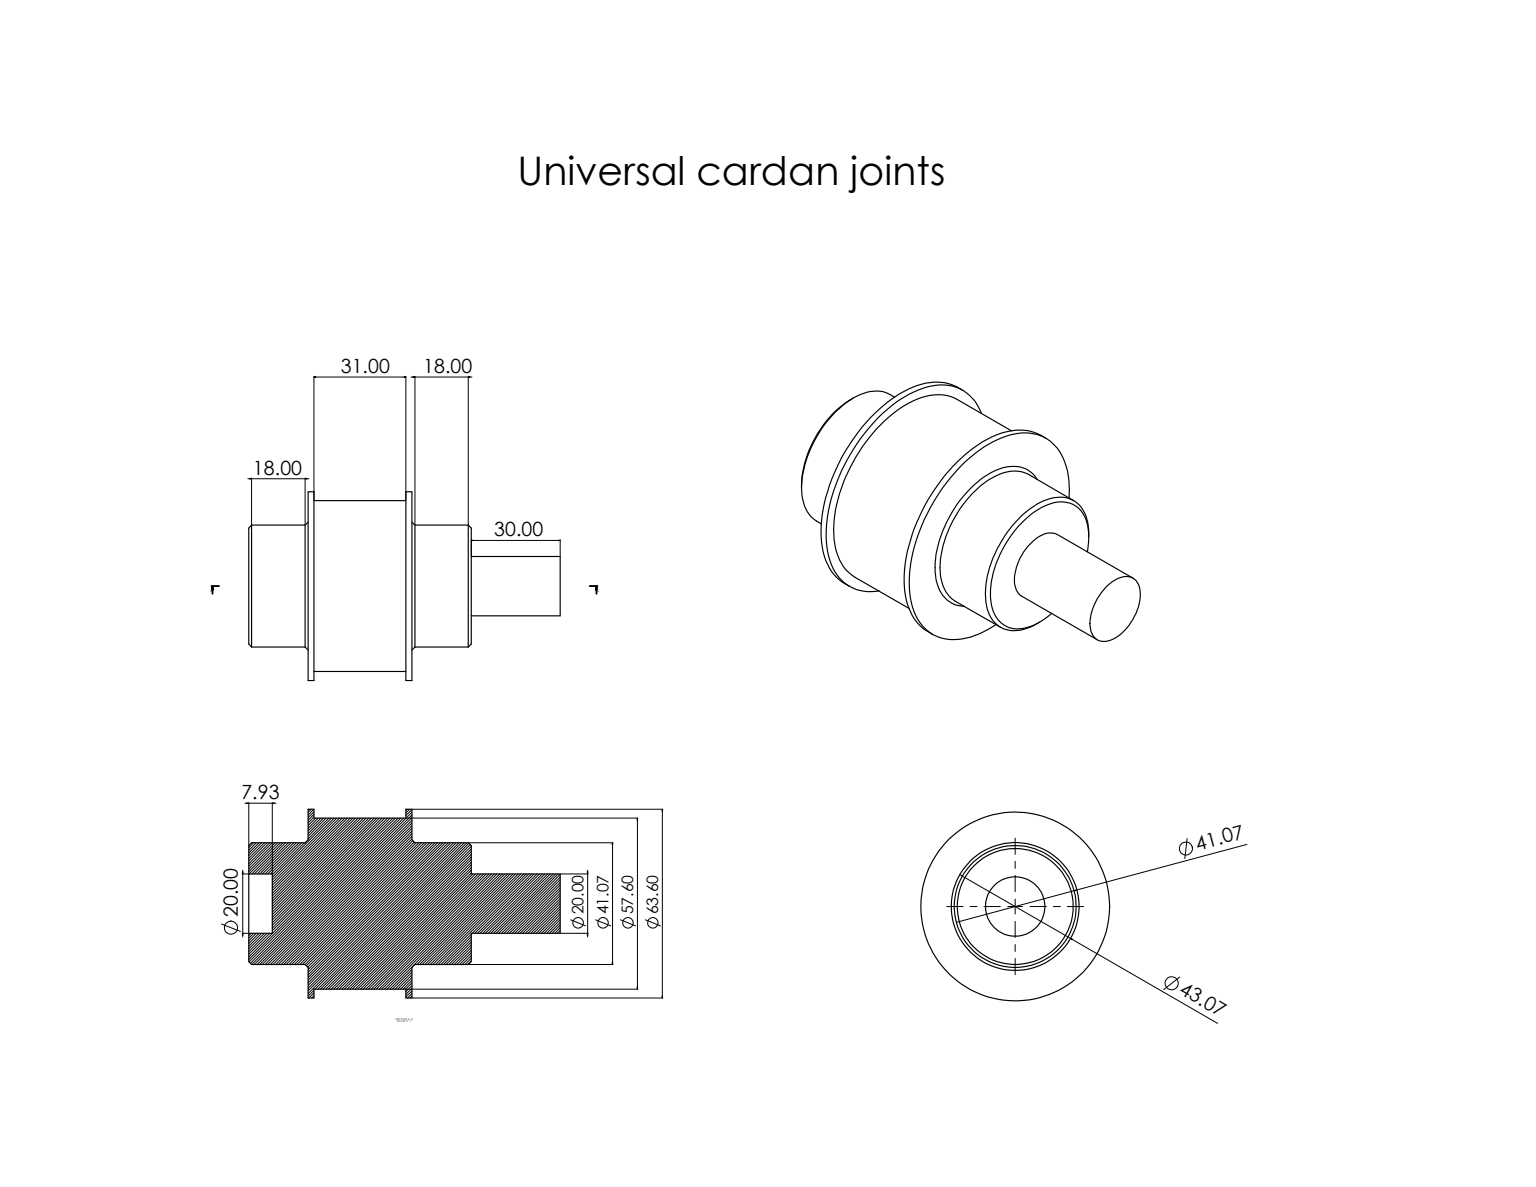
ISO-10303-21;
HEADER;
FILE_DESCRIPTION (('STEP AP214'),
    '1' );
FILE_NAME ('Universal cardan joints.step',
    '2026-10-27T19:20:31',
    ( '' ),
    ( '' ),
    'SwSTEP 2.0',
    'SolidWorks 2025',
    '' );
FILE_SCHEMA (( 'AUTOMOTIVE_DESIGN' ));
ENDSEC;

DATA;
#22=DIRECTION ( 'NONE',  ( 0.000000000000000000, 0.000000000000000000, 1.000000000000000000 ) ) ;
#28=ORIENTED_EDGE ( 'NONE', *, *, #15718, .T. ) ;
#34=DIRECTION ( 'NONE',  ( 0.000000000000000000, 0.000000000000000000, 1.000000000000000000 ) ) ;
#74=DIRECTION ( 'NONE',  ( -1.000000000000000000, 0.000000000000000000, 0.000000000000000000 ) ) ;
#91=ORIENTED_EDGE ( 'NONE', *, *, #1926, .F. ) ;
#97=VECTOR ( 'NONE', #21456, 1000.000000000000000 ) ;
#195=PRODUCT ( 'Universal cardan joints', 'Universal cardan joints', '', ( #26348 ) ) ;
#244=AXIS2_PLACEMENT_3D ( 'NONE', #3180, #21532, #25538 ) ;
#277=AXIS2_PLACEMENT_3D ( 'NONE', #11873, #9385, #1278 ) ;
#288=ORIENTED_EDGE ( 'NONE', *, *, #2639, .F. ) ;
#299=DIRECTION ( 'NONE',  ( -1.000000000000000000, -0.000000000000000000, -0.000000000000000000 ) ) ;
#421=CARTESIAN_POINT ( 'NONE',  ( -370.0000000000001137, -4.857225732735059864E-14, 0.000000000000000000 ) ) ;
#440=CARTESIAN_POINT ( 'NONE',  ( -295.0000000000000568, -4.857225732735059864E-14, 0.000000000000000000 ) ) ;
#464=AXIS2_PLACEMENT_3D ( 'NONE', #3688, #20320, #23901 ) ;
#478=DIRECTION ( 'NONE',  ( 0.000000000000000000, 0.000000000000000000, -1.000000000000000000 ) ) ;
#495=VERTEX_POINT ( 'NONE', #11725 ) ;
#573=DIRECTION ( 'NONE',  ( -1.000000000000000000, 0.000000000000000000, -0.000000000000000000 ) ) ;
#612=ADVANCED_FACE ( 'NONE', ( #6031 ), #23234, .T. ) ;
#783=CARTESIAN_POINT ( 'NONE',  ( -314.0000000000000568, -4.857225732735059864E-14, 0.000000000000000000 ) ) ;
#811=LINE ( 'NONE', #8516, #13626 ) ;
#825=( NAMED_UNIT ( * ) SI_UNIT ( $, .STERADIAN. ) SOLID_ANGLE_UNIT ( ) );
#827=ORIENTED_EDGE ( 'NONE', *, *, #8764, .F. ) ;
#862=VERTEX_POINT ( 'NONE', #20801 ) ;
#941=DIRECTION ( 'NONE',  ( -0.7071067811865302533, 0.000000000000000000, 0.7071067811865646702 ) ) ;
#984=ORIENTED_EDGE ( 'NONE', *, *, #22744, .T. ) ;
#996=DIRECTION ( 'NONE',  ( 0.000000000000000000, 0.000000000000000000, -1.000000000000000000 ) ) ;
#1025=EDGE_CURVE ( 'NONE', #20774, #23054, #12596, .T. ) ;
#1113=ORIENTED_EDGE ( 'NONE', *, *, #21755, .F. ) ;
#1121=PRODUCT_DEFINITION_CONTEXT ( 'detailed design', #16139, 'design' ) ;
#1241=ORIENTED_EDGE ( 'NONE', *, *, #9230, .F. ) ;
#1257=DIRECTION ( 'NONE',  ( 1.000000000000000000, 0.000000000000000000, 0.000000000000000000 ) ) ;
#1278=DIRECTION ( 'NONE',  ( 0.000000000000000000, 0.000000000000000000, -1.000000000000000000 ) ) ;
#1284=PLANE ( 'NONE',  #7860 ) ;
#1298=CARTESIAN_POINT ( 'NONE',  ( -296.0000000000000000, -4.857225732735059864E-14, 0.000000000000000000 ) ) ;
#1340=AXIS2_PLACEMENT_3D ( 'NONE', #8100, #26229, #11702 ) ;
#1341=CARTESIAN_POINT ( 'NONE',  ( -315.0000000000000568, -4.857225732735059864E-14, 0.000000000000000000 ) ) ;
#1377=ORIENTED_EDGE ( 'NONE', *, *, #13860, .T. ) ;
#1381=AXIS2_PLACEMENT_3D ( 'NONE', #11675, #9306, #19800 ) ;
#1389=CARTESIAN_POINT ( 'NONE',  ( -317.0000000000000568, -4.857225732735059864E-14, -31.79780246617542616 ) ) ;
#1404=DIRECTION ( 'NONE',  ( -1.000000000000000000, 0.000000000000000000, 0.000000000000000000 ) ) ;
#1425=VERTEX_POINT ( 'NONE', #2470 ) ;
#1458=DIRECTION ( 'NONE',  ( 0.000000000000000000, 0.000000000000000000, 1.000000000000000000 ) ) ;
#1507=CARTESIAN_POINT ( 'NONE',  ( -317.0000000000000568, -4.857225732735059864E-14, 0.000000000000000000 ) ) ;
#1570=UNCERTAINTY_MEASURE_WITH_UNIT (LENGTH_MEASURE( 1.000000000000000082E-05 ), #17119, 'distance_accuracy_value', 'NONE');
#1574=AXIS2_PLACEMENT_3D ( 'NONE', #23163, #13295, #7298 ) ;
#1578=CARTESIAN_POINT ( 'NONE',  ( -265.0000000000000000, -4.857225732735059864E-14, 10.00000000000000000 ) ) ;
#1579=DIRECTION ( 'NONE',  ( 0.7071067811865500152, 8.659560562354903276E-17, 0.7071067811865451302 ) ) ;
#1608=CARTESIAN_POINT ( 'NONE',  ( -362.0709805440841365, -4.734761052820324085E-14, -10.00000000000004796 ) ) ;
#1686=AXIS2_PLACEMENT_3D ( 'NONE', #17256, #9399, #13145 ) ;
#1695=CARTESIAN_POINT ( 'NONE',  ( -317.0000000000000568, -4.857225732735059864E-14, 0.000000000000000000 ) ) ;
#1704=CARTESIAN_POINT ( 'NONE',  ( -362.0709805440841365, -4.605747634845933236E-14, -20.53474504356812247 ) ) ;
#1740=EDGE_CURVE ( 'NONE', #20774, #862, #9363, .T. ) ;
#1766=AXIS2_PLACEMENT_3D ( 'NONE', #25196, #2714, #11077 ) ;
#1881=CARTESIAN_POINT ( 'NONE',  ( -295.0000000000000568, -4.734761052820324716E-14, -9.999999999999996447 ) ) ;
#1926=EDGE_CURVE ( 'NONE', #1425, #13433, #19253, .T. ) ;
#2016=ADVANCED_FACE ( 'NONE', ( #25514, #21508 ), #1284, .F. ) ;
#2084=AXIS2_PLACEMENT_3D ( 'NONE', #2569, #12809, #10684 ) ;
#2108=CYLINDRICAL_SURFACE ( 'NONE', #18230, 31.79780246617542616 ) ;
#2126=CIRCLE ( 'NONE', #10610, 20.53474504356812247 ) ;
#2127=ORIENTED_EDGE ( 'NONE', *, *, #14586, .T. ) ;
#2190=AXIS2_PLACEMENT_3D ( 'NONE', #6287, #4316, #22000 ) ;
#2213=DIRECTION ( 'NONE',  ( 1.000000000000000000, 0.000000000000000000, 0.000000000000000000 ) ) ;
#2326=LINE ( 'NONE', #18553, #4936 ) ;
#2385=DIRECTION ( 'NONE',  ( 0.000000000000000000, 0.000000000000000000, -1.000000000000000000 ) ) ;
#2390=DIRECTION ( 'NONE',  ( 0.000000000000000000, 0.000000000000000000, 1.000000000000000000 ) ) ;
#2455=VERTEX_POINT ( 'NONE', #6167 ) ;
#2470=CARTESIAN_POINT ( 'NONE',  ( -351.0000000000000568, -4.857225732735059864E-14, 20.53474504356812247 ) ) ;
#2497=AXIS2_PLACEMENT_3D ( 'NONE', #14303, #74, #16164 ) ;
#2564=FACE_OUTER_BOUND ( 'NONE', #16654, .T. ) ;
#2569=CARTESIAN_POINT ( 'NONE',  ( -362.0709805440841365, -4.857225732735059864E-14, 0.000000000000000000 ) ) ;
#2604=VECTOR ( 'NONE', #11874, 1000.000000000000000 ) ;
#2639=EDGE_CURVE ( 'NONE', #19072, #19714, #10510, .T. ) ;
#2697=VERTEX_POINT ( 'NONE', #10914 ) ;
#2709=DIRECTION ( 'NONE',  ( 1.000000000000000000, 0.000000000000000000, 0.000000000000000000 ) ) ;
#2714=DIRECTION ( 'NONE',  ( -1.000000000000000000, 0.000000000000000000, -0.000000000000000000 ) ) ;
#2830=ORIENTED_EDGE ( 'NONE', *, *, #4790, .T. ) ;
#2832=EDGE_LOOP ( 'NONE', ( #20393, #22553, #11090, #13813 ) ) ;
#2980=ADVANCED_FACE ( 'NONE', ( #9043 ), #15154, .F. ) ;
#3049=DIRECTION ( 'NONE',  ( -1.000000000000000000, -0.000000000000000000, -0.000000000000000000 ) ) ;
#3051=AXIS2_PLACEMENT_3D ( 'NONE', #24614, #22620, #12897 ) ;
#3055=DIRECTION ( 'NONE',  ( -1.000000000000000000, 0.000000000000000000, -0.000000000000000000 ) ) ;
#3081=AXIS2_PLACEMENT_3D ( 'NONE', #17412, #7552, #23664 ) ;
#3087=DIRECTION ( 'NONE',  ( -1.000000000000000000, 0.000000000000000000, 0.000000000000000000 ) ) ;
#3107=CARTESIAN_POINT ( 'NONE',  ( -315.0000000000000568, -4.857225732735059864E-14, 21.53474504356810115 ) ) ;
#3118=EDGE_CURVE ( 'NONE', #3897, #22348, #16821, .T. ) ;
#3146=EDGE_CURVE ( 'NONE', #26122, #19577, #26173, .T. ) ;
#3180=CARTESIAN_POINT ( 'NONE',  ( -370.0000000000001137, -4.857225732735059864E-14, 0.000000000000000000 ) ) ;
#3200=ORIENTED_EDGE ( 'NONE', *, *, #9955, .T. ) ;
#3209=CARTESIAN_POINT ( 'NONE',  ( -351.0000000000000568, -4.857225732735059864E-14, 0.000000000000000000 ) ) ;
#3237=CIRCLE ( 'NONE', #18086, 19.53474504356812602 ) ;
#3318=ORIENTED_EDGE ( 'NONE', *, *, #9230, .T. ) ;
#3329=EDGE_LOOP ( 'NONE', ( #14913, #4122, #9477, #25461 ) ) ;
#3365=DIRECTION ( 'NONE',  ( 1.000000000000000000, 0.000000000000000000, 0.000000000000000000 ) ) ;
#3366=VECTOR ( 'NONE', #1579, 1000.000000000000114 ) ;
#3420=ORIENTED_EDGE ( 'NONE', *, *, #7342, .T. ) ;
#3452=EDGE_LOOP ( 'NONE', ( #17676, #18778 ) ) ;
#3466=DIRECTION ( 'NONE',  ( 0.000000000000000000, 0.000000000000000000, -1.000000000000000000 ) ) ;
#3478=FACE_OUTER_BOUND ( 'NONE', #10035, .T. ) ;
#3548=CARTESIAN_POINT ( 'NONE',  ( -317.0000000000000568, -4.857225732735059864E-14, 0.000000000000000000 ) ) ;
#3593=DIRECTION ( 'NONE',  ( 0.000000000000000000, 0.000000000000000000, 1.000000000000000000 ) ) ;
#3615=ORIENTED_EDGE ( 'NONE', *, *, #8737, .F. ) ;
#3629=( GEOMETRIC_REPRESENTATION_CONTEXT ( 3 ) GLOBAL_UNCERTAINTY_ASSIGNED_CONTEXT ( ( #21784 ) ) GLOBAL_UNIT_ASSIGNED_CONTEXT ( ( #17040, #24777, #825 ) ) REPRESENTATION_CONTEXT ( 'NONE', 'WORKASPACE' ) );
#3684=DIRECTION ( 'NONE',  ( 0.000000000000000000, 0.000000000000000000, 1.000000000000000000 ) ) ;
#3688=CARTESIAN_POINT ( 'NONE',  ( -295.0000000000000568, -4.857225732735059864E-14, 0.000000000000000000 ) ) ;
#3789=AXIS2_PLACEMENT_3D ( 'NONE', #16859, #22989, #21124 ) ;
#3812=ADVANCED_FACE ( 'NONE', ( #15407 ), #23532, .T. ) ;
#3897=VERTEX_POINT ( 'NONE', #1578 ) ;
#3913=AXIS2_PLACEMENT_3D ( 'NONE', #9877, #299, #22401 ) ;
#3914=CARTESIAN_POINT ( 'NONE',  ( -317.0000000000000568, -4.857225732735059864E-14, 0.000000000000000000 ) ) ;
#3940=DIRECTION ( 'NONE',  ( 0.000000000000000000, 0.000000000000000000, -1.000000000000000000 ) ) ;
#4072=DIRECTION ( 'NONE',  ( -1.000000000000000000, -0.000000000000000000, -0.000000000000000000 ) ) ;
#4089=VECTOR ( 'NONE', #2213, 1000.000000000000000 ) ;
#4092=ORIENTED_EDGE ( 'NONE', *, *, #18990, .F. ) ;
#4122=ORIENTED_EDGE ( 'NONE', *, *, #21755, .T. ) ;
#4252=CARTESIAN_POINT ( 'NONE',  ( -369.0000000000000568, -4.857225732735059864E-14, 0.000000000000000000 ) ) ;
#4257=VERTEX_POINT ( 'NONE', #14149 ) ;
#4316=DIRECTION ( 'NONE',  ( 1.000000000000000000, 0.000000000000000000, 0.000000000000000000 ) ) ;
#4457=EDGE_CURVE ( 'NONE', #1425, #2455, #2326, .T. ) ;
#4510=DIRECTION ( 'NONE',  ( 1.000000000000000000, 0.000000000000000000, 0.000000000000000000 ) ) ;
#4597=EDGE_CURVE ( 'NONE', #18341, #10496, #17055, .T. ) ;
#4687=ORIENTED_EDGE ( 'NONE', *, *, #15718, .F. ) ;
#4688=VERTEX_POINT ( 'NONE', #9710 ) ;
#4761=DIRECTION ( 'NONE',  ( -1.000000000000000000, 0.000000000000000000, 0.000000000000000000 ) ) ;
#4790=EDGE_CURVE ( 'NONE', #1425, #19072, #15746, .T. ) ;
#4796=FACE_OUTER_BOUND ( 'NONE', #26350, .T. ) ;
#4934=AXIS2_PLACEMENT_3D ( 'NONE', #10843, #11349, #15346 ) ;
#4936=VECTOR ( 'NONE', #14558, 1000.000000000000114 ) ;
#4982=ORIENTED_EDGE ( 'NONE', *, *, #25512, .F. ) ;
#5056=DIRECTION ( 'NONE',  ( -0.000000000000000000, 0.000000000000000000, 1.000000000000000000 ) ) ;
#5070=ORIENTED_EDGE ( 'NONE', *, *, #8188, .T. ) ;
#5071=DIRECTION ( 'NONE',  ( 0.000000000000000000, 0.000000000000000000, -1.000000000000000000 ) ) ;
#5080=ORIENTED_EDGE ( 'NONE', *, *, #11566, .F. ) ;
#5123=CIRCLE ( 'NONE', #19140, 9.999999999999996447 ) ;
#5141=ORIENTED_EDGE ( 'NONE', *, *, #22568, .T. ) ;
#5148=CIRCLE ( 'NONE', #2190, 20.53474504356812247 ) ;
#5195=DIRECTION ( 'NONE',  ( 1.000000000000000000, 0.000000000000000000, 0.000000000000000000 ) ) ;
#5200=ORIENTED_EDGE ( 'NONE', *, *, #7342, .F. ) ;
#5202=CIRCLE ( 'NONE', #23470, 20.53474504356812247 ) ;
#5303=DIRECTION ( 'NONE',  ( 0.000000000000000000, 0.000000000000000000, 1.000000000000000000 ) ) ;
#5311=FACE_BOUND ( 'NONE', #11458, .T. ) ;
#5318=VERTEX_POINT ( 'NONE', #25324 ) ;
#5344=CARTESIAN_POINT ( 'NONE',  ( -362.0709805440841365, -4.857225732735059864E-14, 0.000000000000000000 ) ) ;
#5389=ORIENTED_EDGE ( 'NONE', *, *, #8188, .F. ) ;
#5398=EDGE_CURVE ( 'NONE', #22348, #12615, #22238, .T. ) ;
#5426=CYLINDRICAL_SURFACE ( 'NONE', #10487, 28.79780246617542616 ) ;
#5451=ORIENTED_EDGE ( 'NONE', *, *, #22923, .F. ) ;
#5461=DIRECTION ( 'NONE',  ( 1.000000000000000000, 0.000000000000000000, 0.000000000000000000 ) ) ;
#5462=CARTESIAN_POINT ( 'NONE',  ( -362.0709805440841365, -4.857225732735059864E-14, 0.000000000000000000 ) ) ;
#5484=ORIENTED_EDGE ( 'NONE', *, *, #3118, .F. ) ;
#5557=DIRECTION ( 'NONE',  ( -1.000000000000000000, -0.000000000000000000, -0.000000000000000000 ) ) ;
#5585=AXIS2_PLACEMENT_3D ( 'NONE', #16615, #10501, #10769 ) ;
#5591=CARTESIAN_POINT ( 'NONE',  ( -351.0000000000000568, -4.857225732735059864E-14, 0.000000000000000000 ) ) ;
#5670=ORIENTED_EDGE ( 'NONE', *, *, #25498, .F. ) ;
#5673=DIRECTION ( 'NONE',  ( -1.000000000000000000, 0.000000000000000000, 0.000000000000000000 ) ) ;
#5682=FACE_OUTER_BOUND ( 'NONE', #20386, .T. ) ;
#5695=ORIENTED_EDGE ( 'NONE', *, *, #24587, .F. ) ;
#5753=DIRECTION ( 'NONE',  ( 1.000000000000000000, -0.000000000000000000, -0.000000000000000000 ) ) ;
#5862=DIRECTION ( 'NONE',  ( -1.000000000000000000, -0.000000000000000000, -0.000000000000000000 ) ) ;
#5888=FACE_OUTER_BOUND ( 'NONE', #17196, .T. ) ;
#5970=CIRCLE ( 'NONE', #8460, 31.79780246617542616 ) ;
#6031=FACE_OUTER_BOUND ( 'NONE', #6436, .T. ) ;
#6066=FACE_OUTER_BOUND ( 'NONE', #15547, .T. ) ;
#6088=DIRECTION ( 'NONE',  ( 1.000000000000000000, 0.000000000000000000, 0.000000000000000000 ) ) ;
#6138=DIRECTION ( 'NONE',  ( -0.7071067811865302533, 8.659560562355141167E-17, -0.7071067811865646702 ) ) ;
#6148=ORIENTED_EDGE ( 'NONE', *, *, #22583, .T. ) ;
#6167=CARTESIAN_POINT ( 'NONE',  ( -350.0000000000001137, -4.593501166854460352E-14, 21.53474504356805852 ) ) ;
#6235=ORIENTED_EDGE ( 'NONE', *, *, #18921, .F. ) ;
#6243=EDGE_LOOP ( 'NONE', ( #984, #9603 ) ) ;
#6280=DIRECTION ( 'NONE',  ( -1.000000000000000000, -0.000000000000000000, -0.000000000000000000 ) ) ;
#6287=CARTESIAN_POINT ( 'NONE',  ( -369.0000000000000568, -4.857225732735059864E-14, 0.000000000000000000 ) ) ;
#6336=CARTESIAN_POINT ( 'NONE',  ( -317.0000000000000568, -4.857225732735059864E-14, 0.000000000000000000 ) ) ;
#6343=VECTOR ( 'NONE', #6138, 1000.000000000000114 ) ;
#6399=SHAPE_REPRESENTATION_RELATIONSHIP ( 'NONE' , 'NONE' ,  #21040, #11792 ) ;
#6405=ORIENTED_EDGE ( 'NONE', *, *, #18921, .T. ) ;
#6436=EDGE_LOOP ( 'NONE', ( #22771, #14509, #17547, #288 ) ) ;
#6440=AXIS2_PLACEMENT_3D ( 'NONE', #1341, #17551, #15184 ) ;
#6468=ORIENTED_EDGE ( 'NONE', *, *, #22744, .F. ) ;
#6480=EDGE_CURVE ( 'NONE', #26122, #4257, #18309, .T. ) ;
#6565=ORIENTED_EDGE ( 'NONE', *, *, #16134, .F. ) ;
#6574=DIRECTION ( 'NONE',  ( 0.000000000000000000, 0.000000000000000000, -1.000000000000000000 ) ) ;
#6610=AXIS2_PLACEMENT_3D ( 'NONE', #19276, #5557, #17148 ) ;
#6639=AXIS2_PLACEMENT_3D ( 'NONE', #23295, #5195, #5071 ) ;
#6659=DIRECTION ( 'NONE',  ( -1.000000000000000000, -0.000000000000000000, -0.000000000000000000 ) ) ;
#6675=PLANE ( 'NONE',  #14841 ) ;
#6720=ADVANCED_FACE ( 'NONE', ( #11547 ), #25548, .T. ) ;
#6769=AXIS2_PLACEMENT_3D ( 'NONE', #6336, #22588, #12593 ) ;
#6877=AXIS2_PLACEMENT_3D ( 'NONE', #1695, #9800, #17905 ) ;
#6889=EDGE_LOOP ( 'NONE', ( #827, #7372 ) ) ;
#6922=DIRECTION ( 'NONE',  ( 0.000000000000000000, 0.000000000000000000, 1.000000000000000000 ) ) ;
#6943=PLANE ( 'NONE',  #1766 ) ;
#6970=AXIS2_PLACEMENT_3D ( 'NONE', #3548, #25913, #23896 ) ;
#7029=AXIS2_PLACEMENT_3D ( 'NONE', #15084, #10978, #996 ) ;
#7082=LINE ( 'NONE', #11324, #18554 ) ;
#7094=CARTESIAN_POINT ( 'NONE',  ( -295.0000000000000568, -4.857225732735059864E-14, 0.000000000000000000 ) ) ;
#7104=CIRCLE ( 'NONE', #8369, 19.53474504356807273 ) ;
#7147=ORIENTED_EDGE ( 'NONE', *, *, #11566, .T. ) ;
#7179=EDGE_LOOP ( 'NONE', ( #23041, #11086, #5200, #5080 ) ) ;
#7204=CIRCLE ( 'NONE', #1686, 31.79780246617542616 ) ;
#7226=CIRCLE ( 'NONE', #17824, 31.79780246617542616 ) ;
#7255=EDGE_CURVE ( 'NONE', #12861, #24474, #19694, .T. ) ;
#7268=DIRECTION ( 'NONE',  ( 1.000000000000000000, 0.000000000000000000, 0.000000000000000000 ) ) ;
#7298=DIRECTION ( 'NONE',  ( 0.000000000000000000, 0.000000000000000000, 1.000000000000000000 ) ) ;
#7329=CYLINDRICAL_SURFACE ( 'NONE', #13197, 9.999999999999998224 ) ;
#7342=EDGE_CURVE ( 'NONE', #16610, #19577, #21831, .T. ) ;
#7346=ORIENTED_EDGE ( 'NONE', *, *, #19154, .T. ) ;
#7349=DIRECTION ( 'NONE',  ( 0.000000000000000000, 0.000000000000000000, -1.000000000000000000 ) ) ;
#7372=ORIENTED_EDGE ( 'NONE', *, *, #6480, .F. ) ;
#7385=DIRECTION ( 'NONE',  ( 0.000000000000000000, 0.000000000000000000, -1.000000000000000000 ) ) ;
#7430=ORIENTED_EDGE ( 'NONE', *, *, #21493, .T. ) ;
#7465=CARTESIAN_POINT ( 'NONE',  ( -362.0709805440841365, 10.00000000000000000, 0.000000000000000000 ) ) ;
#7501=CIRCLE ( 'NONE', #1574, 19.53474504356812602 ) ;
#7530=LINE ( 'NONE', #21776, #14536 ) ;
#7545=DIRECTION ( 'NONE',  ( 1.000000000000000000, -0.000000000000000000, -0.000000000000000000 ) ) ;
#7552=DIRECTION ( 'NONE',  ( 1.000000000000000000, 0.000000000000000000, 0.000000000000000000 ) ) ;
#7568=DIRECTION ( 'NONE',  ( 0.000000000000000000, 0.000000000000000000, 1.000000000000000000 ) ) ;
#7573=CYLINDRICAL_SURFACE ( 'NONE', #24715, 10.00000000000004796 ) ;
#7623=VERTEX_POINT ( 'NONE', #7932 ) ;
#7668=CARTESIAN_POINT ( 'NONE',  ( -315.0000000000000568, -4.857225732735059864E-14, -31.79780246617542616 ) ) ;
#7673=DIRECTION ( 'NONE',  ( -1.000000000000000000, -0.000000000000000000, -0.000000000000000000 ) ) ;
#7676=CIRCLE ( 'NONE', #25963, 21.53474504356805852 ) ;
#7704=DIRECTION ( 'NONE',  ( 0.000000000000000000, 0.000000000000000000, -1.000000000000000000 ) ) ;
#7730=ORIENTED_EDGE ( 'NONE', *, *, #13704, .F. ) ;
#7784=VERTEX_POINT ( 'NONE', #14717 ) ;
#7835=DIRECTION ( 'NONE',  ( 0.000000000000000000, 0.000000000000000000, -1.000000000000000000 ) ) ;
#7853=CARTESIAN_POINT ( 'NONE',  ( -315.0000000000000568, -4.467814962633844109E-14, 31.79780246617542616 ) ) ;
#7858=AXIS2_PLACEMENT_3D ( 'NONE', #23843, #5753, #17463 ) ;
#7860=AXIS2_PLACEMENT_3D ( 'NONE', #13138, #9392, #7385 ) ;
#7929=LINE ( 'NONE', #12059, #19617 ) ;
#7932=CARTESIAN_POINT ( 'NONE',  ( -348.0000000000001137, -4.467814962633844109E-14, -31.79780246617542616 ) ) ;
#7994=CARTESIAN_POINT ( 'NONE',  ( 0.000000000000000000, 0.000000000000000000, 0.000000000000000000 ) ) ;
#8033=AXIS2_PLACEMENT_3D ( 'NONE', #19816, #23556, #7568 ) ;
#8040=PRODUCT_DEFINITION_SHAPE ( 'NONE', 'NONE',  #17594 ) ;
#8050=DIRECTION ( 'NONE',  ( 0.000000000000000000, 0.000000000000000000, 1.000000000000000000 ) ) ;
#8100=CARTESIAN_POINT ( 'NONE',  ( -362.0709805440841365, -4.857225732735059864E-14, 0.000000000000000000 ) ) ;
#8112=AXIS2_PLACEMENT_3D ( 'NONE', #5591, #21820, #7704 ) ;
#8178=DIRECTION ( 'NONE',  ( 1.000000000000000000, 0.000000000000000000, 0.000000000000000000 ) ) ;
#8188=EDGE_CURVE ( 'NONE', #13247, #25916, #19618, .T. ) ;
#8224=ORIENTED_EDGE ( 'NONE', *, *, #23857, .F. ) ;
#8330=VECTOR ( 'NONE', #17781, 1000.000000000000000 ) ;
#8366=CARTESIAN_POINT ( 'NONE',  ( -315.0000000000000568, -4.857225732735059864E-14, 0.000000000000000000 ) ) ;
#8367=CARTESIAN_POINT ( 'NONE',  ( -348.0000000000001137, -4.857225732735059864E-14, 0.000000000000000000 ) ) ;
#8369=AXIS2_PLACEMENT_3D ( 'NONE', #15880, #11903, #3940 ) ;
#8460=AXIS2_PLACEMENT_3D ( 'NONE', #9947, #7545, #26207 ) ;
#8516=CARTESIAN_POINT ( 'NONE',  ( -296.0000000000000000, -4.857225732735059864E-14, 20.53474504356812247 ) ) ;
#8544=DIRECTION ( 'NONE',  ( 0.000000000000000000, 0.000000000000000000, 1.000000000000000000 ) ) ;
#8549=VECTOR ( 'NONE', #1404, 1000.000000000000000 ) ;
#8572=AXIS2_PLACEMENT_3D ( 'NONE', #17426, #3087, #13435 ) ;
#8672=ADVANCED_FACE ( 'NONE', ( #15343 ), #18820, .T. ) ;
#8678=DIRECTION ( 'NONE',  ( -0.000000000000000000, 0.000000000000000000, 1.000000000000000000 ) ) ;
#8733=ORIENTED_EDGE ( 'NONE', *, *, #5398, .T. ) ;
#8737=EDGE_CURVE ( 'NONE', #25916, #7784, #24001, .T. ) ;
#8764=EDGE_CURVE ( 'NONE', #4257, #26122, #16803, .T. ) ;
#8891=ORIENTED_EDGE ( 'NONE', *, *, #7255, .F. ) ;
#8953=DIRECTION ( 'NONE',  ( 0.000000000000000000, 0.000000000000000000, 1.000000000000000000 ) ) ;
#9009=EDGE_CURVE ( 'NONE', #5318, #21077, #13405, .T. ) ;
#9043=FACE_OUTER_BOUND ( 'NONE', #3329, .T. ) ;
#9065=CARTESIAN_POINT ( 'NONE',  ( -295.0000000000000568, -4.611870868841669993E-14, -19.53474504356812602 ) ) ;
#9221=DIRECTION ( 'NONE',  ( 1.000000000000000000, 0.000000000000000000, 0.000000000000000000 ) ) ;
#9226=ORIENTED_EDGE ( 'NONE', *, *, #12729, .T. ) ;
#9230=EDGE_CURVE ( 'NONE', #12861, #21077, #20513, .T. ) ;
#9233=CONICAL_SURFACE ( 'NONE', #17237, 19.53474504356807273, 0.7853981633974447263 ) ;
#9253=EDGE_LOOP ( 'NONE', ( #20479, #13421 ) ) ;
#9294=FACE_OUTER_BOUND ( 'NONE', #17839, .T. ) ;
#9306=DIRECTION ( 'NONE',  ( -1.000000000000000000, -0.000000000000000000, -0.000000000000000000 ) ) ;
#9316=ORIENTED_EDGE ( 'NONE', *, *, #3118, .T. ) ;
#9319=CYLINDRICAL_SURFACE ( 'NONE', #8572, 31.79780246617542616 ) ;
#9349=ORIENTED_EDGE ( 'NONE', *, *, #22155, .T. ) ;
#9363=LINE ( 'NONE', #9492, #23198 ) ;
#9368=CIRCLE ( 'NONE', #8033, 20.53474504356812247 ) ;
#9385=DIRECTION ( 'NONE',  ( 1.000000000000000000, 0.000000000000000000, 0.000000000000000000 ) ) ;
#9392=DIRECTION ( 'NONE',  ( -1.000000000000000000, 0.000000000000000000, 0.000000000000000000 ) ) ;
#9399=DIRECTION ( 'NONE',  ( 1.000000000000000000, -0.000000000000000000, -0.000000000000000000 ) ) ;
#9408=DIRECTION ( 'NONE',  ( -1.000000000000000000, -0.000000000000000000, -0.000000000000000000 ) ) ;
#9477=ORIENTED_EDGE ( 'NONE', *, *, #24685, .T. ) ;
#9492=CARTESIAN_POINT ( 'NONE',  ( -370.0000000000001137, -4.857225732735059864E-14, -19.53474504356807273 ) ) ;
#9589=DIRECTION ( 'NONE',  ( 0.000000000000000000, 0.000000000000000000, 1.000000000000000000 ) ) ;
#9603=ORIENTED_EDGE ( 'NONE', *, *, #25512, .T. ) ;
#9607=AXIS2_PLACEMENT_3D ( 'NONE', #3209, #5461, #3466 ) ;
#9710=CARTESIAN_POINT ( 'NONE',  ( -295.0000000000000568, -4.857225732735059864E-14, 9.999999999999996447 ) ) ;
#9800=DIRECTION ( 'NONE',  ( 1.000000000000000000, 0.000000000000000000, 0.000000000000000000 ) ) ;
#9811=DIRECTION ( 'NONE',  ( 0.000000000000000000, 0.000000000000000000, 1.000000000000000000 ) ) ;
#9820=CIRCLE ( 'NONE', #13233, 20.53474504356812247 ) ;
#9828=CARTESIAN_POINT ( 'NONE',  ( -315.0000000000000568, -4.857225732735059864E-14, 0.000000000000000000 ) ) ;
#9877=CARTESIAN_POINT ( 'NONE',  ( -362.0709805440841365, -4.857225732735059864E-14, 0.000000000000000000 ) ) ;
#9947=CARTESIAN_POINT ( 'NONE',  ( -348.0000000000001137, -4.857225732735059864E-14, 0.000000000000000000 ) ) ;
#9955=EDGE_CURVE ( 'NONE', #22348, #3897, #18694, .T. ) ;
#9985=LINE ( 'NONE', #21029, #20451 ) ;
#10035=EDGE_LOOP ( 'NONE', ( #23584, #3200, #25176, #4982 ) ) ;
#10043=CIRCLE ( 'NONE', #21634, 21.53474504356810115 ) ;
#10141=ORIENTED_EDGE ( 'NONE', *, *, #22568, .F. ) ;
#10173=CIRCLE ( 'NONE', #20378, 20.53474504356812247 ) ;
#10217=DIRECTION ( 'NONE',  ( 0.000000000000000000, 0.000000000000000000, 1.000000000000000000 ) ) ;
#10270=ORIENTED_EDGE ( 'NONE', *, *, #1025, .T. ) ;
#10279=CARTESIAN_POINT ( 'NONE',  ( -348.0000000000001137, -4.504554366608264653E-14, -28.79780246617542616 ) ) ;
#10304=ADVANCED_FACE ( 'NONE', ( #12669 ), #20797, .T. ) ;
#10361=ORIENTED_EDGE ( 'NONE', *, *, #13860, .F. ) ;
#10418=VECTOR ( 'NONE', #23747, 1000.000000000000000 ) ;
#10449=CARTESIAN_POINT ( 'NONE',  ( -370.0000000000001137, 20.53474504356807273, 0.000000000000000000 ) ) ;
#10467=CONICAL_SURFACE ( 'NONE', #9607, 20.53474504356812247, 0.7853981633974447263 ) ;
#10487=AXIS2_PLACEMENT_3D ( 'NONE', #13158, #3049, #25659 ) ;
#10496=VERTEX_POINT ( 'NONE', #1608 ) ;
#10497=DIRECTION ( 'NONE',  ( 1.000000000000000000, 0.000000000000000000, 0.000000000000000000 ) ) ;
#10501=DIRECTION ( 'NONE',  ( -1.000000000000000000, -0.000000000000000000, -0.000000000000000000 ) ) ;
#10510=LINE ( 'NONE', #24623, #14254 ) ;
#10522=EDGE_LOOP ( 'NONE', ( #11062, #12001, #18006, #14214 ) ) ;
#10610=AXIS2_PLACEMENT_3D ( 'NONE', #783, #7268, #11020 ) ;
#10654=VECTOR ( 'NONE', #12805, 1000.000000000000000 ) ;
#10681=CARTESIAN_POINT ( 'NONE',  ( -315.0000000000000568, 20.53474504356807273, 0.000000000000000000 ) ) ;
#10684=DIRECTION ( 'NONE',  ( 0.000000000000000000, 0.000000000000000000, 1.000000000000000000 ) ) ;
#10769=DIRECTION ( 'NONE',  ( 0.000000000000000000, 0.000000000000000000, 1.000000000000000000 ) ) ;
#10819=CARTESIAN_POINT ( 'NONE',  ( -369.0000000000000568, -4.857225732735059864E-14, 20.53474504356812247 ) ) ;
#10843=CARTESIAN_POINT ( 'NONE',  ( -362.0709805440841365, -4.857225732735059864E-14, 0.000000000000000000 ) ) ;
#10871=DIRECTION ( 'NONE',  ( 0.000000000000000000, 0.000000000000000000, 1.000000000000000000 ) ) ;
#10914=CARTESIAN_POINT ( 'NONE',  ( -296.0000000000000000, -4.605747634845933236E-14, -20.53474504356812247 ) ) ;
#10959=CARTESIAN_POINT ( 'NONE',  ( -350.0000000000001137, -4.857225732735059864E-14, 0.000000000000000000 ) ) ;
#10978=DIRECTION ( 'NONE',  ( 1.000000000000000000, 0.000000000000000000, 0.000000000000000000 ) ) ;
#11020=DIRECTION ( 'NONE',  ( 0.000000000000000000, 0.000000000000000000, 1.000000000000000000 ) ) ;
#11030=EDGE_CURVE ( 'NONE', #21077, #5318, #13951, .T. ) ;
#11052=ORIENTED_EDGE ( 'NONE', *, *, #9955, .F. ) ;
#11062=ORIENTED_EDGE ( 'NONE', *, *, #4457, .F. ) ;
#11077=DIRECTION ( 'NONE',  ( -0.000000000000000000, 0.000000000000000000, 1.000000000000000000 ) ) ;
#11086=ORIENTED_EDGE ( 'NONE', *, *, #3146, .T. ) ;
#11090=ORIENTED_EDGE ( 'NONE', *, *, #13704, .T. ) ;
#11112=ADVANCED_FACE ( 'NONE', ( #6066, #16300 ), #24561, .F. ) ;
#11124=CONICAL_SURFACE ( 'NONE', #3051, 20.53474504356812247, 0.7853981633974725929 ) ;
#11199=CARTESIAN_POINT ( 'NONE',  ( -265.0000000000000000, -4.734761052820324716E-14, -10.00000000000000000 ) ) ;
#11203=DIRECTION ( 'NONE',  ( 0.000000000000000000, 0.000000000000000000, 1.000000000000000000 ) ) ;
#11204=DIRECTION ( 'NONE',  ( -1.000000000000000000, -0.000000000000000000, -0.000000000000000000 ) ) ;
#11283=AXIS2_PLACEMENT_3D ( 'NONE', #17787, #7673, #5303 ) ;
#11284=CARTESIAN_POINT ( 'NONE',  ( -296.0000000000000000, -4.857225732735059864E-14, 0.000000000000000000 ) ) ;
#11292=AXIS2_PLACEMENT_3D ( 'NONE', #13664, #3055, #5056 ) ;
#11324=CARTESIAN_POINT ( 'NONE',  ( -362.0709805440841365, -4.857225732735059864E-14, 20.53474504356812247 ) ) ;
#11337=FACE_OUTER_BOUND ( 'NONE', #9253, .T. ) ;
#11349=DIRECTION ( 'NONE',  ( -1.000000000000000000, -0.000000000000000000, -0.000000000000000000 ) ) ;
#11437=DIRECTION ( 'NONE',  ( 0.000000000000000000, 0.000000000000000000, 1.000000000000000000 ) ) ;
#11458=EDGE_LOOP ( 'NONE', ( #14554, #17516 ) ) ;
#11462=VERTEX_POINT ( 'NONE', #15727 ) ;
#11542=EDGE_LOOP ( 'NONE', ( #9316, #8733, #6468, #5451 ) ) ;
#11547=FACE_OUTER_BOUND ( 'NONE', #15453, .T. ) ;
#11558=FACE_OUTER_BOUND ( 'NONE', #11542, .T. ) ;
#11566=EDGE_CURVE ( 'NONE', #4257, #16610, #19470, .T. ) ;
#11675=CARTESIAN_POINT ( 'NONE',  ( -370.0000000000001137, -4.857225732735059864E-14, 0.000000000000000000 ) ) ;
#11702=DIRECTION ( 'NONE',  ( 0.000000000000000000, 0.000000000000000000, 1.000000000000000000 ) ) ;
#11714=AXIS2_PLACEMENT_3D ( 'NONE', #24564, #14439, #8050 ) ;
#11721=CARTESIAN_POINT ( 'NONE',  ( -317.0000000000000568, -4.857225732735059864E-14, 0.000000000000000000 ) ) ;
#11725=CARTESIAN_POINT ( 'NONE',  ( -295.0000000000000568, -4.857225732735059864E-14, 19.53474504356812602 ) ) ;
#11792=ADVANCED_BREP_SHAPE_REPRESENTATION ( '', ( #17642, #21058 ), #3629 ) ;
#11800=LINE ( 'NONE', #1704, #8330 ) ;
#11873=CARTESIAN_POINT ( 'NONE',  ( -351.0000000000000568, -4.857225732735059864E-14, 0.000000000000000000 ) ) ;
#11874=DIRECTION ( 'NONE',  ( -1.000000000000000000, -0.000000000000000000, -0.000000000000000000 ) ) ;
#11903=DIRECTION ( 'NONE',  ( -1.000000000000000000, -0.000000000000000000, -0.000000000000000000 ) ) ;
#11950=ORIENTED_EDGE ( 'NONE', *, *, #18331, .F. ) ;
#11965=LINE ( 'NONE', #16350, #22181 ) ;
#11984=CIRCLE ( 'NONE', #6877, 28.79780246617542616 ) ;
#11999=EDGE_CURVE ( 'NONE', #19714, #2455, #7676, .T. ) ;
#12001=ORIENTED_EDGE ( 'NONE', *, *, #20689, .F. ) ;
#12059=CARTESIAN_POINT ( 'NONE',  ( -362.0709805440841365, -4.605747634845933236E-14, -20.53474504356812247 ) ) ;
#12075=DIRECTION ( 'NONE',  ( -1.000000000000000000, 0.000000000000000000, 0.000000000000000000 ) ) ;
#12095=ORIENTED_EDGE ( 'NONE', *, *, #25498, .T. ) ;
#12135=VERTEX_POINT ( 'NONE', #21065 ) ;
#12146=LINE ( 'NONE', #22406, #2604 ) ;
#12237=ADVANCED_FACE ( 'NONE', ( #13453 ), #17825, .T. ) ;
#12487=ORIENTED_EDGE ( 'NONE', *, *, #20689, .T. ) ;
#12516=ORIENTED_EDGE ( 'NONE', *, *, #21493, .F. ) ;
#12568=PRODUCT_DEFINITION_FORMATION_WITH_SPECIFIED_SOURCE ( 'ANY', '', #195, .NOT_KNOWN. ) ;
#12569=DIRECTION ( 'NONE',  ( 1.000000000000000000, 0.000000000000000000, 0.000000000000000000 ) ) ;
#12593=DIRECTION ( 'NONE',  ( 0.000000000000000000, 0.000000000000000000, -1.000000000000000000 ) ) ;
#12596=CIRCLE ( 'NONE', #17269, 19.53474504356807273 ) ;
#12615=VERTEX_POINT ( 'NONE', #1881 ) ;
#12624=ORIENTED_EDGE ( 'NONE', *, *, #22583, .F. ) ;
#12626=FACE_OUTER_BOUND ( 'NONE', #18244, .T. ) ;
#12634=DIRECTION ( 'NONE',  ( 0.7071067811865500152, 0.000000000000000000, -0.7071067811865451302 ) ) ;
#12641=EDGE_CURVE ( 'NONE', #17673, #12135, #9985, .T. ) ;
#12660=ORIENTED_EDGE ( 'NONE', *, *, #17278, .F. ) ;
#12666=CARTESIAN_POINT ( 'NONE',  ( -314.0000000000000568, -4.857225732735059864E-14, 20.53474504356812247 ) ) ;
#12669=FACE_OUTER_BOUND ( 'NONE', #18204, .T. ) ;
#12695=AXIS2_PLACEMENT_3D ( 'NONE', #10449, #12569, #478 ) ;
#12729=EDGE_CURVE ( 'NONE', #495, #18845, #811, .T. ) ;
#12805=DIRECTION ( 'NONE',  ( -1.000000000000000000, -0.000000000000000000, -0.000000000000000000 ) ) ;
#12809=DIRECTION ( 'NONE',  ( -1.000000000000000000, -0.000000000000000000, -0.000000000000000000 ) ) ;
#12861=VERTEX_POINT ( 'NONE', #14270 ) ;
#12897=DIRECTION ( 'NONE',  ( 0.000000000000000000, 0.000000000000000000, 1.000000000000000000 ) ) ;
#13020=ORIENTED_EDGE ( 'NONE', *, *, #15149, .T. ) ;
#13064=EDGE_CURVE ( 'NONE', #18341, #22608, #12146, .T. ) ;
#13068=EDGE_CURVE ( 'NONE', #13433, #862, #5148, .T. ) ;
#13129=ADVANCED_FACE ( 'NONE', ( #14003 ), #18394, .T. ) ;
#13138=CARTESIAN_POINT ( 'NONE',  ( -348.0000000000001137, -4.857225732735059864E-14, 0.000000000000000000 ) ) ;
#13145=DIRECTION ( 'NONE',  ( 0.000000000000000000, 0.000000000000000000, -1.000000000000000000 ) ) ;
#13158=CARTESIAN_POINT ( 'NONE',  ( -362.0709805440841365, -4.857225732735059864E-14, 0.000000000000000000 ) ) ;
#13197=AXIS2_PLACEMENT_3D ( 'NONE', #21328, #11204, #9589 ) ;
#13233=AXIS2_PLACEMENT_3D ( 'NONE', #24450, #6088, #22460 ) ;
#13247=VERTEX_POINT ( 'NONE', #20667 ) ;
#13295=DIRECTION ( 'NONE',  ( 1.000000000000000000, 0.000000000000000000, 0.000000000000000000 ) ) ;
#13334=LINE ( 'NONE', #3107, #97 ) ;
#13346=ADVANCED_FACE ( 'NONE', ( #20802 ), #6943, .F. ) ;
#13376=ADVANCED_FACE ( 'NONE', ( #16796 ), #24933, .T. ) ;
#13405=CIRCLE ( 'NONE', #22779, 28.79780246617542616 ) ;
#13421=ORIENTED_EDGE ( 'NONE', *, *, #16396, .T. ) ;
#13433=VERTEX_POINT ( 'NONE', #10819 ) ;
#13435=DIRECTION ( 'NONE',  ( 0.000000000000000000, 0.000000000000000000, 1.000000000000000000 ) ) ;
#13453=FACE_OUTER_BOUND ( 'NONE', #24480, .T. ) ;
#13567=DIRECTION ( 'NONE',  ( -1.000000000000000000, -0.000000000000000000, -0.000000000000000000 ) ) ;
#13588=ORIENTED_EDGE ( 'NONE', *, *, #7255, .T. ) ;
#13621=CARTESIAN_POINT ( 'NONE',  ( -348.0000000000001137, -4.857225732735059864E-14, 31.79780246617542616 ) ) ;
#13626=VECTOR ( 'NONE', #941, 1000.000000000000114 ) ;
#13658=ADVANCED_FACE ( 'NONE', ( #17686 ), #7573, .F. ) ;
#13664=CARTESIAN_POINT ( 'NONE',  ( -295.0000000000000568, 9.999999999999948486, 0.000000000000000000 ) ) ;
#13704=EDGE_CURVE ( 'NONE', #17673, #22942, #9820, .T. ) ;
#13714=ORIENTED_EDGE ( 'NONE', *, *, #24102, .F. ) ;
#13717=PLANE ( 'NONE',  #18701 ) ;
#13813=ORIENTED_EDGE ( 'NONE', *, *, #14586, .F. ) ;
#13816=DIRECTION ( 'NONE',  ( -1.000000000000000000, -0.000000000000000000, -0.000000000000000000 ) ) ;
#13827=CARTESIAN_POINT ( 'NONE',  ( -370.0000000000001137, -4.857225732735059864E-14, 0.000000000000000000 ) ) ;
#13856=DIRECTION ( 'NONE',  ( 0.000000000000000000, 0.000000000000000000, -1.000000000000000000 ) ) ;
#13860=EDGE_CURVE ( 'NONE', #19577, #16610, #22161, .T. ) ;
#13951=CIRCLE ( 'NONE', #2497, 28.79780246617542616 ) ;
#14003=FACE_OUTER_BOUND ( 'NONE', #15036, .T. ) ;
#14059=AXIS2_PLACEMENT_3D ( 'NONE', #9828, #17931, #1458 ) ;
#14149=CARTESIAN_POINT ( 'NONE',  ( -317.0000000000000568, -4.857225732735059864E-14, -31.79780246617542616 ) ) ;
#14202=FACE_OUTER_BOUND ( 'NONE', #14394, .T. ) ;
#14214=ORIENTED_EDGE ( 'NONE', *, *, #18047, .F. ) ;
#14254=VECTOR ( 'NONE', #12634, 1000.000000000000114 ) ;
#14270=CARTESIAN_POINT ( 'NONE',  ( -317.0000000000000568, -4.504554366608264653E-14, -28.79780246617542616 ) ) ;
#14287=ORIENTED_EDGE ( 'NONE', *, *, #1740, .F. ) ;
#14303=CARTESIAN_POINT ( 'NONE',  ( -348.0000000000001137, -4.857225732735059864E-14, 0.000000000000000000 ) ) ;
#14394=EDGE_LOOP ( 'NONE', ( #10141, #6405, #12095, #5389 ) ) ;
#14439=DIRECTION ( 'NONE',  ( -1.000000000000000000, -0.000000000000000000, -0.000000000000000000 ) ) ;
#14509=ORIENTED_EDGE ( 'NONE', *, *, #4457, .T. ) ;
#14536=VECTOR ( 'NONE', #5673, 1000.000000000000000 ) ;
#14554=ORIENTED_EDGE ( 'NONE', *, *, #11999, .T. ) ;
#14558=DIRECTION ( 'NONE',  ( 0.7071067811865500152, 8.659560562354903276E-17, 0.7071067811865451302 ) ) ;
#14578=CARTESIAN_POINT ( 'NONE',  ( -350.0000000000001137, -4.857225732735059864E-14, -21.53474504356805852 ) ) ;
#14586=EDGE_CURVE ( 'NONE', #18845, #22942, #7082, .T. ) ;
#14709=CLOSED_SHELL ( 'NONE', ( #22016, #6720, #612, #16473, #21026, #2980, #22589, #13376, #21593, #8672, #12237, #15396, #13129, #22165, #13346, #23462, #16453, #3812, #23084, #2016, #21489, #25442, #13658, #11112, #10304, #18234, #16295, #16957, #21985, #17209 ) ) ;
#14717=CARTESIAN_POINT ( 'NONE',  ( -350.0000000000001137, -4.467814962633844109E-14, -31.79780246617542616 ) ) ;
#14841=AXIS2_PLACEMENT_3D ( 'NONE', #10681, #573, #8678 ) ;
#14908=ORIENTED_EDGE ( 'NONE', *, *, #24102, .T. ) ;
#14913=ORIENTED_EDGE ( 'NONE', *, *, #16396, .F. ) ;
#14921=CARTESIAN_POINT ( 'NONE',  ( -362.0709805440841365, -4.857225732735059864E-14, 9.999999999999998224 ) ) ;
#15012=ORIENTED_EDGE ( 'NONE', *, *, #19065, .F. ) ;
#15036=EDGE_LOOP ( 'NONE', ( #21580, #22914, #7147, #10361 ) ) ;
#15084=CARTESIAN_POINT ( 'NONE',  ( -317.0000000000000568, -4.857225732735059864E-14, 0.000000000000000000 ) ) ;
#15149=EDGE_CURVE ( 'NONE', #495, #20259, #7501, .T. ) ;
#15154=CYLINDRICAL_SURFACE ( 'NONE', #6610, 10.00000000000004796 ) ;
#15184=DIRECTION ( 'NONE',  ( 0.000000000000000000, 0.000000000000000000, 1.000000000000000000 ) ) ;
#15317=DIRECTION ( 'NONE',  ( -1.000000000000000000, -0.000000000000000000, -0.000000000000000000 ) ) ;
#15338=ORIENTED_EDGE ( 'NONE', *, *, #12641, .F. ) ;
#15343=FACE_OUTER_BOUND ( 'NONE', #7179, .T. ) ;
#15346=DIRECTION ( 'NONE',  ( 0.000000000000000000, 0.000000000000000000, 1.000000000000000000 ) ) ;
#15396=ADVANCED_FACE ( 'NONE', ( #25150 ), #5426, .T. ) ;
#15407=FACE_OUTER_BOUND ( 'NONE', #26291, .T. ) ;
#15453=EDGE_LOOP ( 'NONE', ( #7730, #15640, #12516, #22475 ) ) ;
#15529=CONICAL_SURFACE ( 'NONE', #19792, 20.53474504356812247, 0.7853981633974725929 ) ;
#15536=PLANE ( 'NONE',  #3081 ) ;
#15547=EDGE_LOOP ( 'NONE', ( #10270, #28 ) ) ;
#15557=FACE_OUTER_BOUND ( 'NONE', #10522, .T. ) ;
#15580=DIRECTION ( 'NONE',  ( 0.000000000000000000, 0.000000000000000000, -1.000000000000000000 ) ) ;
#15640=ORIENTED_EDGE ( 'NONE', *, *, #12641, .T. ) ;
#15647=VECTOR ( 'NONE', #1257, 1000.000000000000000 ) ;
#15701=ORIENTED_EDGE ( 'NONE', *, *, #1740, .T. ) ;
#15707=ORIENTED_EDGE ( 'NONE', *, *, #23136, .F. ) ;
#15718=EDGE_CURVE ( 'NONE', #23054, #20774, #7104, .T. ) ;
#15727=CARTESIAN_POINT ( 'NONE',  ( -315.0000000000000568, -4.857225732735059864E-14, 21.53474504356810115 ) ) ;
#15746=CIRCLE ( 'NONE', #8112, 20.53474504356812247 ) ;
#15759=CARTESIAN_POINT ( 'NONE',  ( -370.0000000000001137, -4.857225732735059864E-14, -19.53474504356807273 ) ) ;
#15880=CARTESIAN_POINT ( 'NONE',  ( -370.0000000000001137, -4.857225732735059864E-14, 0.000000000000000000 ) ) ;
#15977=DIRECTION ( 'NONE',  ( 1.000000000000000000, 0.000000000000000000, 0.000000000000000000 ) ) ;
#16061=CARTESIAN_POINT ( 'NONE',  ( -348.0000000000001137, -4.857225732735059864E-14, 0.000000000000000000 ) ) ;
#16118=EDGE_LOOP ( 'NONE', ( #4687, #6148, #8224, #14287 ) ) ;
#16124=DIRECTION ( 'NONE',  ( -1.000000000000000000, -0.000000000000000000, -0.000000000000000000 ) ) ;
#16134=EDGE_CURVE ( 'NONE', #24474, #5318, #16689, .T. ) ;
#16139=APPLICATION_CONTEXT ( 'automotive_design' ) ;
#16164=DIRECTION ( 'NONE',  ( 0.000000000000000000, 0.000000000000000000, 1.000000000000000000 ) ) ;
#16295=ADVANCED_FACE ( 'NONE', ( #18688 ), #9233, .T. ) ;
#16300=FACE_BOUND ( 'NONE', #16522, .T. ) ;
#16350=CARTESIAN_POINT ( 'NONE',  ( -362.0709805440841365, -4.734761052820324085E-14, -10.00000000000004796 ) ) ;
#16379=ORIENTED_EDGE ( 'NONE', *, *, #16134, .T. ) ;
#16392=CYLINDRICAL_SURFACE ( 'NONE', #3913, 20.53474504356812247 ) ;
#16396=EDGE_CURVE ( 'NONE', #10496, #18341, #21978, .T. ) ;
#16403=DIRECTION ( 'NONE',  ( 0.000000000000000000, 0.000000000000000000, -1.000000000000000000 ) ) ;
#16413=MECHANICAL_DESIGN_GEOMETRIC_PRESENTATION_REPRESENTATION('',(#18539),#20677);
#16453=ADVANCED_FACE ( 'NONE', ( #9294, #23280 ), #23651, .F. ) ;
#16473=ADVANCED_FACE ( 'NONE', ( #25791 ), #20656, .T. ) ;
#16522=EDGE_LOOP ( 'NONE', ( #11950, #26193 ) ) ;
#16610=VERTEX_POINT ( 'NONE', #7668 ) ;
#16615=CARTESIAN_POINT ( 'NONE',  ( -315.0000000000000568, -4.857225732735059864E-14, 0.000000000000000000 ) ) ;
#16654=EDGE_LOOP ( 'NONE', ( #3420, #1377 ) ) ;
#16689=LINE ( 'NONE', #18283, #25342 ) ;
#16712=ORIENTED_EDGE ( 'NONE', *, *, #8737, .T. ) ;
#16733=DIRECTION ( 'NONE',  ( 0.000000000000000000, 0.000000000000000000, -1.000000000000000000 ) ) ;
#16786=EDGE_CURVE ( 'NONE', #20259, #495, #3237, .T. ) ;
#16796=FACE_OUTER_BOUND ( 'NONE', #2832, .T. ) ;
#16800=DIRECTION ( 'NONE',  ( 0.000000000000000000, 0.000000000000000000, -1.000000000000000000 ) ) ;
#16803=CIRCLE ( 'NONE', #18508, 31.79780246617542616 ) ;
#16821=CIRCLE ( 'NONE', #11714, 10.00000000000000000 ) ;
#16859=CARTESIAN_POINT ( 'NONE',  ( -315.0000000000000568, -4.857225732735059864E-14, 0.000000000000000000 ) ) ;
#16910=CARTESIAN_POINT ( 'NONE',  ( -362.0709805440841365, -4.504554366608264653E-14, -28.79780246617542616 ) ) ;
#16957=ADVANCED_FACE ( 'NONE', ( #15557 ), #10467, .T. ) ;
#16986=( NAMED_UNIT ( * ) PLANE_ANGLE_UNIT ( ) SI_UNIT ( $, .RADIAN. ) );
#17040=( LENGTH_UNIT ( ) NAMED_UNIT ( * ) SI_UNIT ( .MILLI., .METRE. ) );
#17055=CIRCLE ( 'NONE', #20452, 10.00000000000004796 ) ;
#17119=( LENGTH_UNIT ( ) NAMED_UNIT ( * ) SI_UNIT ( .MILLI., .METRE. ) );
#17148=DIRECTION ( 'NONE',  ( 0.000000000000000000, 0.000000000000000000, 1.000000000000000000 ) ) ;
#17196=EDGE_LOOP ( 'NONE', ( #2830, #7346, #25815, #91 ) ) ;
#17209=ADVANCED_FACE ( 'NONE', ( #5682 ), #15529, .T. ) ;
#17237=AXIS2_PLACEMENT_3D ( 'NONE', #18420, #8178, #6574 ) ;
#17256=CARTESIAN_POINT ( 'NONE',  ( -348.0000000000001137, -4.857225732735059864E-14, 0.000000000000000000 ) ) ;
#17269=AXIS2_PLACEMENT_3D ( 'NONE', #13827, #24224, #7835 ) ;
#17278=EDGE_CURVE ( 'NONE', #2697, #17673, #11800, .T. ) ;
#17412=CARTESIAN_POINT ( 'NONE',  ( -350.0000000000001137, 20.53474504356807273, 0.000000000000000000 ) ) ;
#17426=CARTESIAN_POINT ( 'NONE',  ( -348.0000000000001137, -4.857225732735059864E-14, 0.000000000000000000 ) ) ;
#17463=DIRECTION ( 'NONE',  ( 0.000000000000000000, 0.000000000000000000, -1.000000000000000000 ) ) ;
#17483=ORIENTED_EDGE ( 'NONE', *, *, #15149, .F. ) ;
#17516=ORIENTED_EDGE ( 'NONE', *, *, #18047, .T. ) ;
#17547=ORIENTED_EDGE ( 'NONE', *, *, #11999, .F. ) ;
#17551=DIRECTION ( 'NONE',  ( -1.000000000000000000, -0.000000000000000000, -0.000000000000000000 ) ) ;
#17594=PRODUCT_DEFINITION ( 'UNKNOWN', '', #12568, #1121 ) ;
#17642=MANIFOLD_SOLID_BREP ( 'Chamfer1', #14709 ) ;
#17673=VERTEX_POINT ( 'NONE', #23251 ) ;
#17676=ORIENTED_EDGE ( 'NONE', *, *, #9009, .T. ) ;
#17686=FACE_OUTER_BOUND ( 'NONE', #19849, .T. ) ;
#17728=APPLICATION_CONTEXT ( 'automotive_design' ) ;
#17768=ORIENTED_EDGE ( 'NONE', *, *, #23947, .T. ) ;
#17781=DIRECTION ( 'NONE',  ( -1.000000000000000000, -0.000000000000000000, -0.000000000000000000 ) ) ;
#17787=CARTESIAN_POINT ( 'NONE',  ( -362.0709805440841365, -4.857225732735059864E-14, 0.000000000000000000 ) ) ;
#17800=EDGE_LOOP ( 'NONE', ( #1241, #15012, #16379, #21140 ) ) ;
#17801=ORIENTED_EDGE ( 'NONE', *, *, #1926, .T. ) ;
#17824=AXIS2_PLACEMENT_3D ( 'NONE', #21842, #25593, #23704 ) ;
#17825=CYLINDRICAL_SURFACE ( 'NONE', #17864, 28.79780246617542616 ) ;
#17834=DIRECTION ( 'NONE',  ( 0.000000000000000000, 0.000000000000000000, -1.000000000000000000 ) ) ;
#17839=EDGE_LOOP ( 'NONE', ( #13020, #22817 ) ) ;
#17864=AXIS2_PLACEMENT_3D ( 'NONE', #5344, #23953, #11203 ) ;
#17898=CONICAL_SURFACE ( 'NONE', #5585, 21.53474504356810115, 0.7853981633974378429 ) ;
#17905=DIRECTION ( 'NONE',  ( 0.000000000000000000, 0.000000000000000000, -1.000000000000000000 ) ) ;
#17922=CARTESIAN_POINT ( 'NONE',  ( -370.0000000000001137, -4.617994102837407382E-14, 19.53474504356807273 ) ) ;
#17931=DIRECTION ( 'NONE',  ( -1.000000000000000000, -0.000000000000000000, -0.000000000000000000 ) ) ;
#17964=ORIENTED_EDGE ( 'NONE', *, *, #23136, .T. ) ;
#18006=ORIENTED_EDGE ( 'NONE', *, *, #2639, .T. ) ;
#18047=EDGE_CURVE ( 'NONE', #2455, #19714, #18113, .T. ) ;
#18086=AXIS2_PLACEMENT_3D ( 'NONE', #440, #2709, #8544 ) ;
#18104=LINE ( 'NONE', #24375, #6343 ) ;
#18113=CIRCLE ( 'NONE', #6639, 21.53474504356805852 ) ;
#18204=EDGE_LOOP ( 'NONE', ( #21342, #12487, #17801, #24282 ) ) ;
#18206=CYLINDRICAL_SURFACE ( 'NONE', #1340, 9.999999999999998224 ) ;
#18230=AXIS2_PLACEMENT_3D ( 'NONE', #16061, #12075, #10217 ) ;
#18234=ADVANCED_FACE ( 'NONE', ( #5311, #25675 ), #15536, .F. ) ;
#18244=EDGE_LOOP ( 'NONE', ( #15338, #13714, #23088, #21488 ) ) ;
#18246=CARTESIAN_POINT ( 'NONE',  ( -351.0000000000000568, -4.857225732735059864E-14, 0.000000000000000000 ) ) ;
#18283=CARTESIAN_POINT ( 'NONE',  ( -362.0709805440841365, -4.857225732735059864E-14, 28.79780246617542616 ) ) ;
#18309=CIRCLE ( 'NONE', #19589, 31.79780246617542616 ) ;
#18331=EDGE_CURVE ( 'NONE', #22608, #20012, #18347, .T. ) ;
#18341=VERTEX_POINT ( 'NONE', #19667 ) ;
#18347=CIRCLE ( 'NONE', #1381, 10.00000000000004796 ) ;
#18394=CYLINDRICAL_SURFACE ( 'NONE', #20875, 31.79780246617542616 ) ;
#18420=CARTESIAN_POINT ( 'NONE',  ( -370.0000000000001137, -4.857225732735059864E-14, 0.000000000000000000 ) ) ;
#18508=AXIS2_PLACEMENT_3D ( 'NONE', #1507, #3365, #7349 ) ;
#18539=STYLED_ITEM('',(#26409),#17642);
#18553=CARTESIAN_POINT ( 'NONE',  ( -351.0000000000000568, -4.605747634845933236E-14, 20.53474504356812247 ) ) ;
#18554=VECTOR ( 'NONE', #15317, 1000.000000000000000 ) ;
#18584=FACE_OUTER_BOUND ( 'NONE', #6889, .T. ) ;
#18609=ORIENTED_EDGE ( 'NONE', *, *, #4597, .F. ) ;
#18688=FACE_OUTER_BOUND ( 'NONE', #22915, .T. ) ;
#18694=CIRCLE ( 'NONE', #21615, 10.00000000000000000 ) ;
#18701=AXIS2_PLACEMENT_3D ( 'NONE', #7465, #9221, #15580 ) ;
#18776=CARTESIAN_POINT ( 'NONE',  ( -350.0000000000001137, -4.857225732735059864E-14, 31.79780246617542616 ) ) ;
#18778=ORIENTED_EDGE ( 'NONE', *, *, #11030, .T. ) ;
#18820=CYLINDRICAL_SURFACE ( 'NONE', #7029, 31.79780246617542616 ) ;
#18845=VERTEX_POINT ( 'NONE', #19331 ) ;
#18912=ORIENTED_EDGE ( 'NONE', *, *, #24587, .T. ) ;
#18921=EDGE_CURVE ( 'NONE', #7623, #7784, #7530, .T. ) ;
#18990=EDGE_CURVE ( 'NONE', #18845, #2697, #5202, .T. ) ;
#19054=LINE ( 'NONE', #14921, #10654 ) ;
#19065=EDGE_CURVE ( 'NONE', #24474, #12861, #11984, .T. ) ;
#19072=VERTEX_POINT ( 'NONE', #24032 ) ;
#19140=AXIS2_PLACEMENT_3D ( 'NONE', #7094, #21457, #23335 ) ;
#19154=EDGE_CURVE ( 'NONE', #19072, #862, #7929, .T. ) ;
#19191=CARTESIAN_POINT ( 'NONE',  ( -362.0709805440841365, -4.857225732735059864E-14, 0.000000000000000000 ) ) ;
#19253=LINE ( 'NONE', #21384, #10418 ) ;
#19276=CARTESIAN_POINT ( 'NONE',  ( -362.0709805440841365, -4.857225732735059864E-14, 0.000000000000000000 ) ) ;
#19331=CARTESIAN_POINT ( 'NONE',  ( -296.0000000000000000, -4.857225732735059864E-14, 20.53474504356812247 ) ) ;
#19470=LINE ( 'NONE', #1389, #15647 ) ;
#19475=EDGE_CURVE ( 'NONE', #22942, #11462, #13334, .T. ) ;
#19553=FACE_OUTER_BOUND ( 'NONE', #20421, .T. ) ;
#19577=VERTEX_POINT ( 'NONE', #7853 ) ;
#19589=AXIS2_PLACEMENT_3D ( 'NONE', #11721, #22607, #17834 ) ;
#19617=VECTOR ( 'NONE', #26189, 1000.000000000000000 ) ;
#19618=LINE ( 'NONE', #13621, #8549 ) ;
#19667=CARTESIAN_POINT ( 'NONE',  ( -362.0709805440841365, -4.857225732735059864E-14, 10.00000000000004796 ) ) ;
#19694=CIRCLE ( 'NONE', #6970, 28.79780246617542616 ) ;
#19714=VERTEX_POINT ( 'NONE', #14578 ) ;
#19791=LINE ( 'NONE', #17922, #3366 ) ;
#19792=AXIS2_PLACEMENT_3D ( 'NONE', #11284, #21923, #9811 ) ;
#19800=DIRECTION ( 'NONE',  ( 0.000000000000000000, 0.000000000000000000, 1.000000000000000000 ) ) ;
#19816=CARTESIAN_POINT ( 'NONE',  ( -296.0000000000000000, -4.857225732735059864E-14, 0.000000000000000000 ) ) ;
#19818=VECTOR ( 'NONE', #5862, 1000.000000000000000 ) ;
#19849=EDGE_LOOP ( 'NONE', ( #1113, #18609, #24473, #21304 ) ) ;
#19989=CIRCLE ( 'NONE', #464, 9.999999999999996447 ) ;
#20012=VERTEX_POINT ( 'NONE', #26120 ) ;
#20103=CARTESIAN_POINT ( 'NONE',  ( -362.0709805440841365, -4.734761052820324716E-14, -9.999999999999998224 ) ) ;
#20133=DIRECTION ( 'NONE',  ( 1.000000000000000000, 0.000000000000000000, 0.000000000000000000 ) ) ;
#20259=VERTEX_POINT ( 'NONE', #9065 ) ;
#20320=DIRECTION ( 'NONE',  ( -1.000000000000000000, -0.000000000000000000, -0.000000000000000000 ) ) ;
#20378=AXIS2_PLACEMENT_3D ( 'NONE', #4252, #4510, #16733 ) ;
#20386=EDGE_LOOP ( 'NONE', ( #5695, #17483, #9226, #15707 ) ) ;
#20393=ORIENTED_EDGE ( 'NONE', *, *, #18990, .T. ) ;
#20421=EDGE_LOOP ( 'NONE', ( #6235, #21590, #5070, #16712 ) ) ;
#20435=CARTESIAN_POINT ( 'NONE',  ( -317.0000000000000568, -4.467814962633844109E-14, 31.79780246617542616 ) ) ;
#20447=AXIS2_PLACEMENT_3D ( 'NONE', #18246, #6280, #13856 ) ;
#20451=VECTOR ( 'NONE', #21163, 1000.000000000000000 ) ;
#20452=AXIS2_PLACEMENT_3D ( 'NONE', #5462, #23559, #11437 ) ;
#20479=ORIENTED_EDGE ( 'NONE', *, *, #4597, .T. ) ;
#20513=LINE ( 'NONE', #16910, #24025 ) ;
#20614=DIRECTION ( 'NONE',  ( -1.000000000000000000, -0.000000000000000000, -0.000000000000000000 ) ) ;
#20656=CONICAL_SURFACE ( 'NONE', #244, 19.53474504356807273, 0.7853981633974447263 ) ;
#20667=CARTESIAN_POINT ( 'NONE',  ( -348.0000000000001137, -4.857225732735059864E-14, 31.79780246617542616 ) ) ;
#20677=( GEOMETRIC_REPRESENTATION_CONTEXT ( 3 ) GLOBAL_UNCERTAINTY_ASSIGNED_CONTEXT ( ( #1570 ) ) GLOBAL_UNIT_ASSIGNED_CONTEXT ( ( #17119, #16986, #22990 ) ) REPRESENTATION_CONTEXT ( 'NONE', 'WORKASPACE' ) );
#20689=EDGE_CURVE ( 'NONE', #19072, #1425, #21312, .T. ) ;
#20723=PLANE ( 'NONE',  #6769 ) ;
#20774=VERTEX_POINT ( 'NONE', #15759 ) ;
#20793=FACE_BOUND ( 'NONE', #23428, .T. ) ;
#20797=CYLINDRICAL_SURFACE ( 'NONE', #2084, 20.53474504356812247 ) ;
#20801=CARTESIAN_POINT ( 'NONE',  ( -369.0000000000000568, -4.605747634845933236E-14, -20.53474504356812247 ) ) ;
#20802=FACE_OUTER_BOUND ( 'NONE', #23512, .T. ) ;
#20875=AXIS2_PLACEMENT_3D ( 'NONE', #3914, #20133, #16403 ) ;
#20891=AXIS2_PLACEMENT_3D ( 'NONE', #19191, #22667, #8953 ) ;
#20928=CARTESIAN_POINT ( 'NONE',  ( -370.0000000000001137, -4.611870868841670624E-14, 19.53474504356807273 ) ) ;
#21008=CARTESIAN_POINT ( 'NONE',  ( -315.0000000000000568, -4.857225732735059864E-14, 0.000000000000000000 ) ) ;
#21026=ADVANCED_FACE ( 'NONE', ( #5888 ), #16392, .T. ) ;
#21029=CARTESIAN_POINT ( 'NONE',  ( -315.0000000000000568, -4.593501166854459721E-14, -21.53474504356810115 ) ) ;
#21040=SHAPE_REPRESENTATION ( 'Universal cardan joints', ( #21058 ), #3629 ) ;
#21058=AXIS2_PLACEMENT_3D ( 'NONE', #7994, #22, #15977 ) ;
#21065=CARTESIAN_POINT ( 'NONE',  ( -315.0000000000000568, -4.593501166854459721E-14, -21.53474504356810115 ) ) ;
#21077=VERTEX_POINT ( 'NONE', #10279 ) ;
#21124=DIRECTION ( 'NONE',  ( 0.000000000000000000, 0.000000000000000000, -1.000000000000000000 ) ) ;
#21140=ORIENTED_EDGE ( 'NONE', *, *, #11030, .F. ) ;
#21163=DIRECTION ( 'NONE',  ( -0.7071067811865549002, 8.659560562354844111E-17, -0.7071067811865401342 ) ) ;
#21304=ORIENTED_EDGE ( 'NONE', *, *, #18331, .T. ) ;
#21310=ORIENTED_EDGE ( 'NONE', *, *, #12729, .F. ) ;
#21312=CIRCLE ( 'NONE', #20447, 20.53474504356812247 ) ;
#21328=CARTESIAN_POINT ( 'NONE',  ( -362.0709805440841365, -4.857225732735059864E-14, 0.000000000000000000 ) ) ;
#21342=ORIENTED_EDGE ( 'NONE', *, *, #19154, .F. ) ;
#21384=CARTESIAN_POINT ( 'NONE',  ( -362.0709805440841365, -4.857225732735059864E-14, 20.53474504356812247 ) ) ;
#21456=DIRECTION ( 'NONE',  ( -0.7071067811865549002, 0.000000000000000000, 0.7071067811865401342 ) ) ;
#21457=DIRECTION ( 'NONE',  ( -1.000000000000000000, -0.000000000000000000, -0.000000000000000000 ) ) ;
#21488=ORIENTED_EDGE ( 'NONE', *, *, #22155, .F. ) ;
#21489=ADVANCED_FACE ( 'NONE', ( #19553 ), #9319, .T. ) ;
#21493=EDGE_CURVE ( 'NONE', #11462, #12135, #23450, .T. ) ;
#21508=FACE_BOUND ( 'NONE', #3452, .T. ) ;
#21532=DIRECTION ( 'NONE',  ( 1.000000000000000000, 0.000000000000000000, 0.000000000000000000 ) ) ;
#21540=AXIS2_PLACEMENT_3D ( 'NONE', #21008, #10497, #2385 ) ;
#21580=ORIENTED_EDGE ( 'NONE', *, *, #3146, .F. ) ;
#21590=ORIENTED_EDGE ( 'NONE', *, *, #23947, .F. ) ;
#21593=ADVANCED_FACE ( 'NONE', ( #11558 ), #18206, .T. ) ;
#21615=AXIS2_PLACEMENT_3D ( 'NONE', #26129, #16124, #34 ) ;
#21634=AXIS2_PLACEMENT_3D ( 'NONE', #8366, #20614, #2390 ) ;
#21642=EDGE_LOOP ( 'NONE', ( #25856, #13588 ) ) ;
#21755=EDGE_CURVE ( 'NONE', #10496, #20012, #11965, .T. ) ;
#21776=CARTESIAN_POINT ( 'NONE',  ( -348.0000000000001137, -4.467814962633844109E-14, -31.79780246617542616 ) ) ;
#21784=UNCERTAINTY_MEASURE_WITH_UNIT (LENGTH_MEASURE( 1.000000000000000082E-05 ), #17040, 'distance_accuracy_value', 'NONE');
#21820=DIRECTION ( 'NONE',  ( -1.000000000000000000, -0.000000000000000000, -0.000000000000000000 ) ) ;
#21831=CIRCLE ( 'NONE', #21540, 31.79780246617542616 ) ;
#21842=CARTESIAN_POINT ( 'NONE',  ( -350.0000000000001137, -4.857225732735059864E-14, 0.000000000000000000 ) ) ;
#21923=DIRECTION ( 'NONE',  ( -1.000000000000000000, -0.000000000000000000, -0.000000000000000000 ) ) ;
#21978=CIRCLE ( 'NONE', #4934, 10.00000000000004796 ) ;
#21985=ADVANCED_FACE ( 'NONE', ( #12626 ), #17898, .T. ) ;
#22000=DIRECTION ( 'NONE',  ( 0.000000000000000000, 0.000000000000000000, -1.000000000000000000 ) ) ;
#22016=ADVANCED_FACE ( 'NONE', ( #4796 ), #11124, .T. ) ;
#22155=EDGE_CURVE ( 'NONE', #12135, #11462, #10043, .T. ) ;
#22161=CIRCLE ( 'NONE', #3789, 31.79780246617542616 ) ;
#22165=ADVANCED_FACE ( 'NONE', ( #24580, #18584 ), #20723, .F. ) ;
#22181=VECTOR ( 'NONE', #13816, 1000.000000000000000 ) ;
#22238=LINE ( 'NONE', #20103, #19818 ) ;
#22348=VERTEX_POINT ( 'NONE', #11199 ) ;
#22392=ORIENTED_EDGE ( 'NONE', *, *, #1025, .F. ) ;
#22401=DIRECTION ( 'NONE',  ( 0.000000000000000000, 0.000000000000000000, 1.000000000000000000 ) ) ;
#22406=CARTESIAN_POINT ( 'NONE',  ( -362.0709805440841365, -4.857225732735059864E-14, 10.00000000000004796 ) ) ;
#22460=DIRECTION ( 'NONE',  ( 0.000000000000000000, 0.000000000000000000, 1.000000000000000000 ) ) ;
#22475=ORIENTED_EDGE ( 'NONE', *, *, #19475, .F. ) ;
#22517=DIRECTION ( 'NONE',  ( -1.000000000000000000, -0.000000000000000000, -0.000000000000000000 ) ) ;
#22553=ORIENTED_EDGE ( 'NONE', *, *, #17278, .T. ) ;
#22568=EDGE_CURVE ( 'NONE', #7623, #13247, #5970, .T. ) ;
#22583=EDGE_CURVE ( 'NONE', #23054, #13433, #19791, .T. ) ;
#22588=DIRECTION ( 'NONE',  ( 1.000000000000000000, 0.000000000000000000, 0.000000000000000000 ) ) ;
#22589=ADVANCED_FACE ( 'NONE', ( #14202 ), #2108, .T. ) ;
#22607=DIRECTION ( 'NONE',  ( 1.000000000000000000, 0.000000000000000000, 0.000000000000000000 ) ) ;
#22608=VERTEX_POINT ( 'NONE', #25797 ) ;
#22620=DIRECTION ( 'NONE',  ( -1.000000000000000000, -0.000000000000000000, -0.000000000000000000 ) ) ;
#22647=ORIENTED_EDGE ( 'NONE', *, *, #16786, .F. ) ;
#22667=DIRECTION ( 'NONE',  ( -1.000000000000000000, -0.000000000000000000, -0.000000000000000000 ) ) ;
#22744=EDGE_CURVE ( 'NONE', #4688, #12615, #19989, .T. ) ;
#22771=ORIENTED_EDGE ( 'NONE', *, *, #4790, .F. ) ;
#22779=AXIS2_PLACEMENT_3D ( 'NONE', #8367, #4761, #10871 ) ;
#22817=ORIENTED_EDGE ( 'NONE', *, *, #16786, .T. ) ;
#22914=ORIENTED_EDGE ( 'NONE', *, *, #6480, .T. ) ;
#22915=EDGE_LOOP ( 'NONE', ( #12624, #22392, #15701, #25750 ) ) ;
#22923=EDGE_CURVE ( 'NONE', #3897, #4688, #19054, .T. ) ;
#22942=VERTEX_POINT ( 'NONE', #12666 ) ;
#22989=DIRECTION ( 'NONE',  ( 1.000000000000000000, 0.000000000000000000, 0.000000000000000000 ) ) ;
#22990=( NAMED_UNIT ( * ) SI_UNIT ( $, .STERADIAN. ) SOLID_ANGLE_UNIT ( ) );
#23041=ORIENTED_EDGE ( 'NONE', *, *, #8764, .T. ) ;
#23054=VERTEX_POINT ( 'NONE', #20928 ) ;
#23084=ADVANCED_FACE ( 'NONE', ( #20793, #2564 ), #6675, .F. ) ;
#23086=ORIENTED_EDGE ( 'NONE', *, *, #9009, .F. ) ;
#23088=ORIENTED_EDGE ( 'NONE', *, *, #19475, .T. ) ;
#23136=EDGE_CURVE ( 'NONE', #2697, #18845, #9368, .T. ) ;
#23163=CARTESIAN_POINT ( 'NONE',  ( -295.0000000000000568, -4.857225732735059864E-14, 0.000000000000000000 ) ) ;
#23198=VECTOR ( 'NONE', #25486, 1000.000000000000114 ) ;
#23234=CONICAL_SURFACE ( 'NONE', #277, 20.53474504356812247, 0.7853981633974447263 ) ;
#23251=CARTESIAN_POINT ( 'NONE',  ( -314.0000000000000568, -4.605747634845933236E-14, -20.53474504356812247 ) ) ;
#23280=FACE_BOUND ( 'NONE', #6243, .T. ) ;
#23295=CARTESIAN_POINT ( 'NONE',  ( -350.0000000000001137, -4.857225732735059864E-14, 0.000000000000000000 ) ) ;
#23298=CARTESIAN_POINT ( 'NONE',  ( -317.0000000000000568, -4.467814962633844109E-14, 31.79780246617542616 ) ) ;
#23335=DIRECTION ( 'NONE',  ( 0.000000000000000000, 0.000000000000000000, 1.000000000000000000 ) ) ;
#23428=EDGE_LOOP ( 'NONE', ( #7430, #9349 ) ) ;
#23450=CIRCLE ( 'NONE', #6440, 21.53474504356810115 ) ;
#23462=ADVANCED_FACE ( 'NONE', ( #3478 ), #7329, .T. ) ;
#23470=AXIS2_PLACEMENT_3D ( 'NONE', #1298, #9408, #3684 ) ;
#23512=EDGE_LOOP ( 'NONE', ( #5484, #11052 ) ) ;
#23532=CYLINDRICAL_SURFACE ( 'NONE', #11283, 20.53474504356812247 ) ;
#23556=DIRECTION ( 'NONE',  ( -1.000000000000000000, -0.000000000000000000, -0.000000000000000000 ) ) ;
#23559=DIRECTION ( 'NONE',  ( -1.000000000000000000, -0.000000000000000000, -0.000000000000000000 ) ) ;
#23584=ORIENTED_EDGE ( 'NONE', *, *, #5398, .F. ) ;
#23651=PLANE ( 'NONE',  #11292 ) ;
#23664=DIRECTION ( 'NONE',  ( 0.000000000000000000, 0.000000000000000000, -1.000000000000000000 ) ) ;
#23704=DIRECTION ( 'NONE',  ( 0.000000000000000000, 0.000000000000000000, -1.000000000000000000 ) ) ;
#23747=DIRECTION ( 'NONE',  ( -1.000000000000000000, -0.000000000000000000, -0.000000000000000000 ) ) ;
#23843=CARTESIAN_POINT ( 'NONE',  ( -350.0000000000001137, -4.857225732735059864E-14, 0.000000000000000000 ) ) ;
#23857=EDGE_CURVE ( 'NONE', #862, #13433, #10173, .T. ) ;
#23896=DIRECTION ( 'NONE',  ( 0.000000000000000000, 0.000000000000000000, -1.000000000000000000 ) ) ;
#23901=DIRECTION ( 'NONE',  ( 0.000000000000000000, 0.000000000000000000, 1.000000000000000000 ) ) ;
#23924=SHAPE_DEFINITION_REPRESENTATION ( #8040, #21040 ) ;
#23947=EDGE_CURVE ( 'NONE', #13247, #7623, #7204, .T. ) ;
#23953=DIRECTION ( 'NONE',  ( -1.000000000000000000, -0.000000000000000000, -0.000000000000000000 ) ) ;
#24001=CIRCLE ( 'NONE', #7858, 31.79780246617542616 ) ;
#24025=VECTOR ( 'NONE', #22517, 1000.000000000000000 ) ;
#24032=CARTESIAN_POINT ( 'NONE',  ( -351.0000000000000568, -4.605747634845933236E-14, -20.53474504356812247 ) ) ;
#24102=EDGE_CURVE ( 'NONE', #22942, #17673, #2126, .T. ) ;
#24224=DIRECTION ( 'NONE',  ( -1.000000000000000000, -0.000000000000000000, -0.000000000000000000 ) ) ;
#24281=EDGE_LOOP ( 'NONE', ( #3615, #5670 ) ) ;
#24282=ORIENTED_EDGE ( 'NONE', *, *, #13068, .T. ) ;
#24324=CARTESIAN_POINT ( 'NONE',  ( -362.0709805440841365, -4.857225732735059864E-14, 0.000000000000000000 ) ) ;
#24375=CARTESIAN_POINT ( 'NONE',  ( -296.0000000000000000, -4.605747634845933236E-14, -20.53474504356812247 ) ) ;
#24450=CARTESIAN_POINT ( 'NONE',  ( -314.0000000000000568, -4.857225732735059864E-14, 0.000000000000000000 ) ) ;
#24473=ORIENTED_EDGE ( 'NONE', *, *, #13064, .T. ) ;
#24474=VERTEX_POINT ( 'NONE', #25745 ) ;
#24480=EDGE_LOOP ( 'NONE', ( #8891, #3318, #23086, #6565 ) ) ;
#24561=PLANE ( 'NONE',  #12695 ) ;
#24564=CARTESIAN_POINT ( 'NONE',  ( -265.0000000000000000, -4.857225732735059864E-14, 0.000000000000000000 ) ) ;
#24580=FACE_BOUND ( 'NONE', #21642, .T. ) ;
#24587=EDGE_CURVE ( 'NONE', #20259, #2697, #18104, .T. ) ;
#24614=CARTESIAN_POINT ( 'NONE',  ( -296.0000000000000000, -4.857225732735059864E-14, 0.000000000000000000 ) ) ;
#24623=CARTESIAN_POINT ( 'NONE',  ( -351.0000000000000568, -4.857225732735059864E-14, -20.53474504356812247 ) ) ;
#24640=CIRCLE ( 'NONE', #25087, 10.00000000000004796 ) ;
#24685=EDGE_CURVE ( 'NONE', #20012, #22608, #24640, .T. ) ;
#24715=AXIS2_PLACEMENT_3D ( 'NONE', #24324, #13567, #3593 ) ;
#24777=( NAMED_UNIT ( * ) PLANE_ANGLE_UNIT ( ) SI_UNIT ( $, .RADIAN. ) );
#24933=CYLINDRICAL_SURFACE ( 'NONE', #20891, 20.53474504356812247 ) ;
#25087=AXIS2_PLACEMENT_3D ( 'NONE', #421, #6659, #6922 ) ;
#25150=FACE_OUTER_BOUND ( 'NONE', #17800, .T. ) ;
#25176=ORIENTED_EDGE ( 'NONE', *, *, #22923, .T. ) ;
#25196=CARTESIAN_POINT ( 'NONE',  ( -265.0000000000000000, -4.857225732735059864E-14, 0.000000000000000000 ) ) ;
#25200=DIRECTION ( 'NONE',  ( 1.000000000000000000, 0.000000000000000000, 0.000000000000000000 ) ) ;
#25324=CARTESIAN_POINT ( 'NONE',  ( -348.0000000000001137, -4.857225732735059864E-14, 28.79780246617542616 ) ) ;
#25342=VECTOR ( 'NONE', #4072, 1000.000000000000000 ) ;
#25442=ADVANCED_FACE ( 'NONE', ( #11337 ), #13717, .F. ) ;
#25461=ORIENTED_EDGE ( 'NONE', *, *, #13064, .F. ) ;
#25486=DIRECTION ( 'NONE',  ( 0.7071067811865500152, 0.000000000000000000, -0.7071067811865451302 ) ) ;
#25498=EDGE_CURVE ( 'NONE', #7784, #25916, #7226, .T. ) ;
#25512=EDGE_CURVE ( 'NONE', #12615, #4688, #5123, .T. ) ;
#25514=FACE_OUTER_BOUND ( 'NONE', #25559, .T. ) ;
#25538=DIRECTION ( 'NONE',  ( 0.000000000000000000, 0.000000000000000000, -1.000000000000000000 ) ) ;
#25548=CONICAL_SURFACE ( 'NONE', #14059, 21.53474504356810115, 0.7853981633974378429 ) ;
#25559=EDGE_LOOP ( 'NONE', ( #17768, #5141 ) ) ;
#25593=DIRECTION ( 'NONE',  ( 1.000000000000000000, -0.000000000000000000, -0.000000000000000000 ) ) ;
#25659=DIRECTION ( 'NONE',  ( 0.000000000000000000, 0.000000000000000000, 1.000000000000000000 ) ) ;
#25675=FACE_OUTER_BOUND ( 'NONE', #24281, .T. ) ;
#25745=CARTESIAN_POINT ( 'NONE',  ( -317.0000000000000568, -4.857225732735059864E-14, 28.79780246617542616 ) ) ;
#25750=ORIENTED_EDGE ( 'NONE', *, *, #13068, .F. ) ;
#25791=FACE_OUTER_BOUND ( 'NONE', #16118, .T. ) ;
#25797=CARTESIAN_POINT ( 'NONE',  ( -370.0000000000001137, -4.857225732735059864E-14, 10.00000000000004796 ) ) ;
#25815=ORIENTED_EDGE ( 'NONE', *, *, #23857, .T. ) ;
#25856=ORIENTED_EDGE ( 'NONE', *, *, #19065, .T. ) ;
#25913=DIRECTION ( 'NONE',  ( 1.000000000000000000, 0.000000000000000000, 0.000000000000000000 ) ) ;
#25916=VERTEX_POINT ( 'NONE', #18776 ) ;
#25963=AXIS2_PLACEMENT_3D ( 'NONE', #10959, #25200, #16800 ) ;
#26120=CARTESIAN_POINT ( 'NONE',  ( -370.0000000000001137, -4.734761052820324085E-14, -10.00000000000004796 ) ) ;
#26122=VERTEX_POINT ( 'NONE', #23298 ) ;
#26129=CARTESIAN_POINT ( 'NONE',  ( -265.0000000000000000, -4.857225732735059864E-14, 0.000000000000000000 ) ) ;
#26173=LINE ( 'NONE', #20435, #4089 ) ;
#26189=DIRECTION ( 'NONE',  ( -1.000000000000000000, -0.000000000000000000, -0.000000000000000000 ) ) ;
#26193=ORIENTED_EDGE ( 'NONE', *, *, #24685, .F. ) ;
#26207=DIRECTION ( 'NONE',  ( 0.000000000000000000, 0.000000000000000000, -1.000000000000000000 ) ) ;
#26229=DIRECTION ( 'NONE',  ( -1.000000000000000000, -0.000000000000000000, -0.000000000000000000 ) ) ;
#26291=EDGE_LOOP ( 'NONE', ( #12660, #17964, #2127, #14908 ) ) ;
#26348=PRODUCT_CONTEXT ( 'NONE', #17728, 'mechanical' ) ;
#26350=EDGE_LOOP ( 'NONE', ( #22647, #18912, #4092, #21310 ) ) ;
#26403=COLOUR_RGB('Off White',0.89,0.88,0.83);
#26404=FILL_AREA_STYLE_COLOUR('',#26403);
#26405=FILL_AREA_STYLE('',(#26404));
#26406=SURFACE_STYLE_FILL_AREA(#26405);
#26407=SURFACE_SIDE_STYLE('',(#26406));
#26408=SURFACE_STYLE_USAGE(.BOTH.,#26407);
#26409=PRESENTATION_STYLE_ASSIGNMENT((#26408));
ENDSEC;
END-ISO-10303-21;
